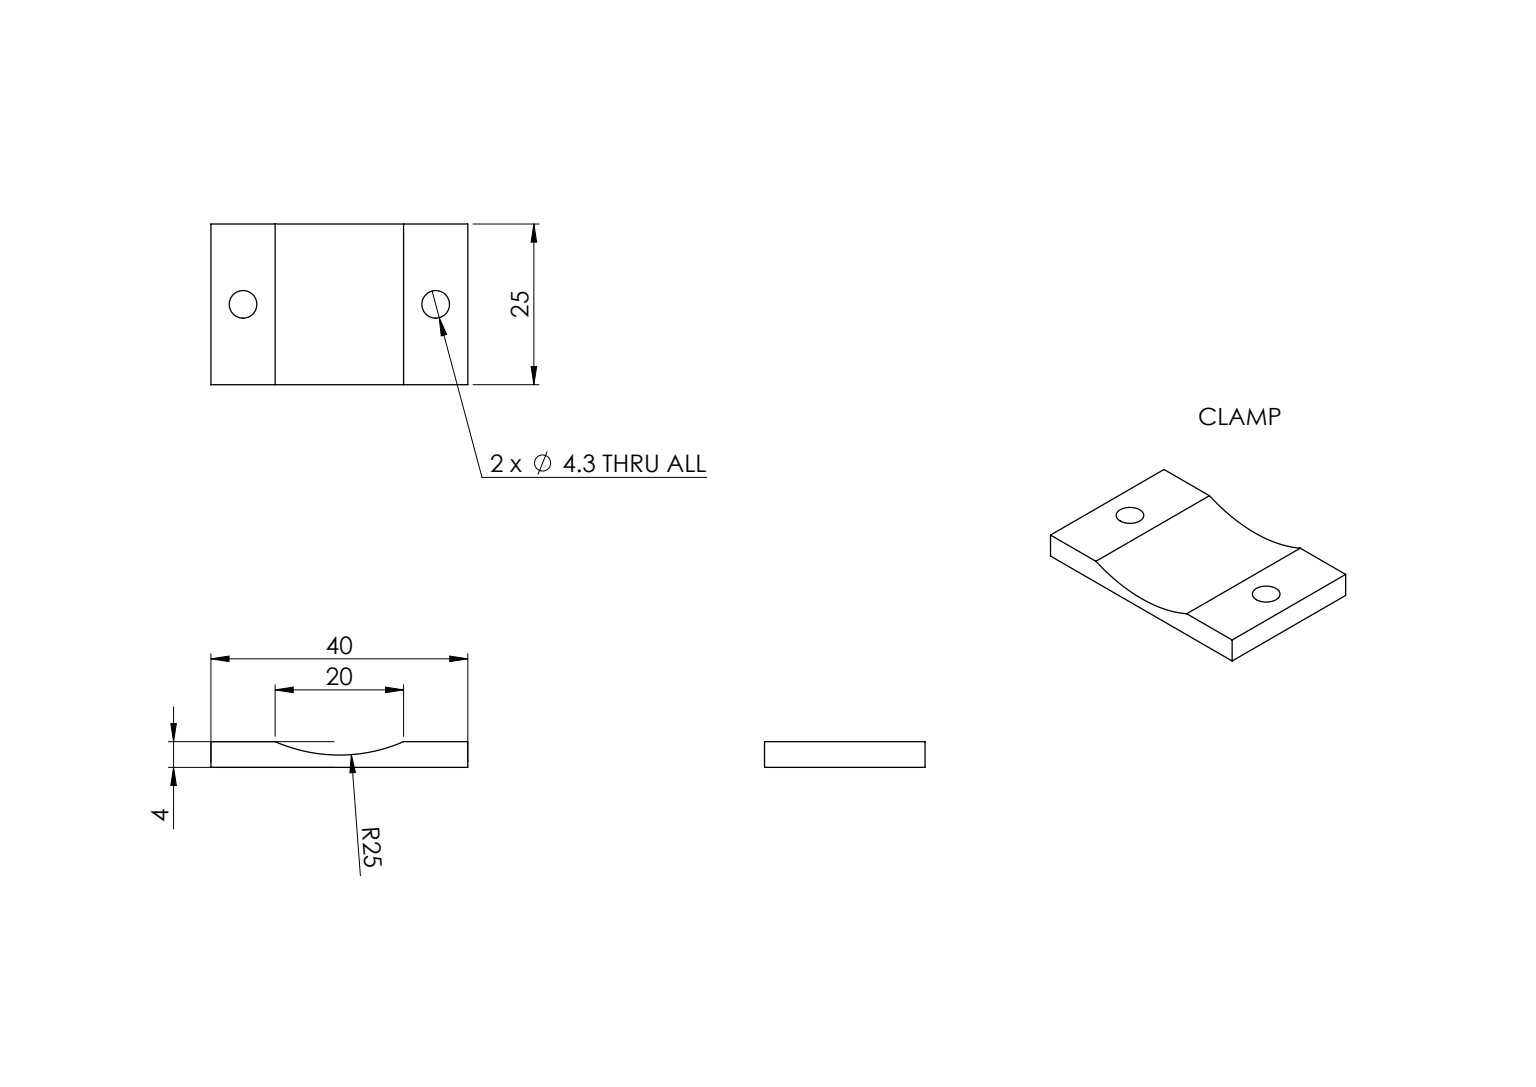
ISO-10303-21;
HEADER;
FILE_DESCRIPTION (('STEP AP214'),
    '1' );
FILE_NAME ('clamp.step',
    '2026-10-27T08:02:39',
    ( '' ),
    ( '' ),
    'SwSTEP 2.0',
    'SolidWorks 2026',
    '' );
FILE_SCHEMA (( 'AUTOMOTIVE_DESIGN' ));
ENDSEC;

DATA;
#6=PLANE ( 'NONE',  #3841 ) ;
#21=( GEOMETRIC_REPRESENTATION_CONTEXT ( 3 ) GLOBAL_UNCERTAINTY_ASSIGNED_CONTEXT ( ( #3529 ) ) GLOBAL_UNIT_ASSIGNED_CONTEXT ( ( #3001, #9758, #2180 ) ) REPRESENTATION_CONTEXT ( 'NONE', 'WORKASPACE' ) );
#33=SHAPE_DEFINITION_REPRESENTATION ( #1615, #7946 ) ;
#110=FACE_OUTER_BOUND ( 'NONE', #7615, .T. ) ;
#120=EDGE_LOOP ( 'NONE', ( #9318, #12086, #3898, #6255 ) ) ;
#123=ORIENTED_EDGE ( 'NONE', *, *, #7333, .T. ) ;
#156=ORIENTED_EDGE ( 'NONE', *, *, #8748, .T. ) ;
#164=CARTESIAN_POINT ( 'NONE',  ( 10.00000000000000000, 44.00000000000001421, -12.50000000000000000 ) ) ;
#182=SURFACE_STYLE_USAGE ( .BOTH. , #5944 ) ;
#191=EDGE_CURVE ( 'NONE', #922, #11041, #11147, .T. ) ;
#200=DIRECTION ( 'NONE',  ( 0.000000000000000000, 0.000000000000000000, 1.000000000000000000 ) ) ;
#212=CARTESIAN_POINT ( 'NONE',  ( 0.000000000000000000, 0.000000000000000000, 0.000000000000000000 ) ) ;
#250=FILL_AREA_STYLE ('',( #6001 ) ) ;
#268=LINE ( 'NONE', #2137, #3626 ) ;
#310=DIRECTION ( 'NONE',  ( 0.000000000000000000, 0.000000000000000000, 1.000000000000000000 ) ) ;
#380=AXIS2_PLACEMENT_3D ( 'NONE', #8436, #6808, #10487 ) ;
#381=ORIENTED_EDGE ( 'NONE', *, *, #191, .T. ) ;
#428=AXIS2_PLACEMENT_3D ( 'NONE', #10140, #7338, #1516 ) ;
#454=AXIS2_PLACEMENT_3D ( 'NONE', #10757, #4010, #11636 ) ;
#455=ORIENTED_EDGE ( 'NONE', *, *, #11034, .T. ) ;
#482=ORIENTED_EDGE ( 'NONE', *, *, #7502, .T. ) ;
#501=DIRECTION ( 'NONE',  ( -0.000000000000000000, 1.000000000000000000, -0.000000000000000000 ) ) ;
#540=ORIENTED_EDGE ( 'NONE', *, *, #2766, .F. ) ;
#557=CARTESIAN_POINT ( 'NONE',  ( -20.00000000000000000, 40.00000000000000711, 12.50000000000000000 ) ) ;
#575=LINE ( 'NONE', #164, #4417 ) ;
#622=LINE ( 'NONE', #3508, #9651 ) ;
#696=LINE ( 'NONE', #8326, #6294 ) ;
#751=DIRECTION ( 'NONE',  ( 0.000000000000000000, -1.000000000000000000, 0.000000000000000000 ) ) ;
#775=EDGE_CURVE ( 'NONE', #5859, #1347, #8071, .T. ) ;
#802=EDGE_LOOP ( 'NONE', ( #5664, #1167, #12118, #8865 ) ) ;
#827=CARTESIAN_POINT ( 'NONE',  ( -20.00000000000000000, 44.00000000000001421, -12.50000000000000000 ) ) ;
#833=EDGE_LOOP ( 'NONE', ( #9307, #5030, #4044, #11673 ) ) ;
#873=CARTESIAN_POINT ( 'NONE',  ( -20.00000000000000000, 44.00000000000001421, -12.50000000000000000 ) ) ;
#880=LINE ( 'NONE', #2008, #11470 ) ;
#922=VERTEX_POINT ( 'NONE', #4486 ) ;
#938=DIRECTION ( 'NONE',  ( 1.000000000000000000, 1.734723475976807094E-16, 0.000000000000000000 ) ) ;
#948=FACE_OUTER_BOUND ( 'NONE', #120, .T. ) ;
#958=LINE ( 'NONE', #4848, #8432 ) ;
#963=ORIENTED_EDGE ( 'NONE', *, *, #1656, .T. ) ;
#981=PLANE ( 'NONE',  #380 ) ;
#988=PLANE ( 'NONE',  #3703 ) ;
#1008=DIRECTION ( 'NONE',  ( 0.000000000000000000, 0.000000000000000000, -1.000000000000000000 ) ) ;
#1011=DIRECTION ( 'NONE',  ( -0.000000000000000000, 0.000000000000000000, -1.000000000000000000 ) ) ;
#1085=PLANE ( 'NONE',  #3231 ) ;
#1093=CARTESIAN_POINT ( 'NONE',  ( 15.00000000000000355, 44.00000000000001421, 2.149999999999999023 ) ) ;
#1104=EDGE_LOOP ( 'NONE', ( #1748, #5954 ) ) ;
#1106=LINE ( 'NONE', #4917, #10396 ) ;
#1119=EDGE_CURVE ( 'NONE', #1183, #3700, #1106, .T. ) ;
#1167=ORIENTED_EDGE ( 'NONE', *, *, #4711, .F. ) ;
#1183=VERTEX_POINT ( 'NONE', #2155 ) ;
#1197=CARTESIAN_POINT ( 'NONE',  ( -15.00000000000000000, 40.00000000000000711, -2.149999999999999023 ) ) ;
#1253=PRODUCT_DEFINITION_FORMATION_WITH_SPECIFIED_SOURCE ( 'ANY', '', #5415, .NOT_KNOWN. ) ;
#1276=DIRECTION ( 'NONE',  ( -0.000000000000000000, 1.000000000000000000, -0.000000000000000000 ) ) ;
#1281=CARTESIAN_POINT ( 'NONE',  ( -15.00000000000000000, 44.00000000000001421, 2.149999999999999023 ) ) ;
#1347=VERTEX_POINT ( 'NONE', #9237 ) ;
#1379=PRODUCT_DEFINITION_CONTEXT ( 'detailed design', #11353, 'design' ) ;
#1516=DIRECTION ( 'NONE',  ( 0.000000000000000000, 0.000000000000000000, 1.000000000000000000 ) ) ;
#1524=DIRECTION ( 'NONE',  ( 0.000000000000000000, 0.000000000000000000, 1.000000000000000000 ) ) ;
#1529=DIRECTION ( 'NONE',  ( -0.000000000000000000, -0.000000000000000000, -1.000000000000000000 ) ) ;
#1539=EDGE_LOOP ( 'NONE', ( #8919, #12318 ) ) ;
#1559=ORIENTED_EDGE ( 'NONE', *, *, #8748, .F. ) ;
#1615=PRODUCT_DEFINITION_SHAPE ( 'NONE', 'NONE',  #5170 ) ;
#1617=ORIENTED_EDGE ( 'NONE', *, *, #3552, .F. ) ;
#1626=CARTESIAN_POINT ( 'NONE',  ( -20.00000000000000000, 44.00000000000001421, 12.50000000000000000 ) ) ;
#1632=ORIENTED_EDGE ( 'NONE', *, *, #9751, .F. ) ;
#1656=EDGE_CURVE ( 'NONE', #5033, #7872, #6765, .T. ) ;
#1714=DIRECTION ( 'NONE',  ( -0.000000000000000000, 1.000000000000000000, -0.000000000000000000 ) ) ;
#1719=EDGE_CURVE ( 'NONE', #10717, #10090, #7363, .T. ) ;
#1739=DIRECTION ( 'NONE',  ( 0.000000000000000000, 0.000000000000000000, -1.000000000000000000 ) ) ;
#1748=ORIENTED_EDGE ( 'NONE', *, *, #4711, .T. ) ;
#1789=EDGE_CURVE ( 'NONE', #8068, #9485, #9216, .T. ) ;
#1851=CARTESIAN_POINT ( 'NONE',  ( 20.00000000000000000, 40.00000000000001421, 12.50000000000000000 ) ) ;
#1952=PLANE ( 'NONE',  #7605 ) ;
#1961=ADVANCED_FACE ( 'NONE', ( #10318 ), #1952, .F. ) ;
#1974=AXIS2_PLACEMENT_3D ( 'NONE', #6094, #1276, #5963 ) ;
#2008=CARTESIAN_POINT ( 'NONE',  ( -20.00000000000000000, 40.00000000000000711, 12.50000000000000000 ) ) ;
#2022=DIRECTION ( 'NONE',  ( 0.000000000000000000, 0.000000000000000000, 1.000000000000000000 ) ) ;
#2137=CARTESIAN_POINT ( 'NONE',  ( 20.00000000000000000, 44.00000000000002132, 12.50000000000000000 ) ) ;
#2155=CARTESIAN_POINT ( 'NONE',  ( -20.00000000000000000, 44.00000000000001421, 12.50000000000000000 ) ) ;
#2180=( NAMED_UNIT ( * ) SI_UNIT ( $, .STERADIAN. ) SOLID_ANGLE_UNIT ( ) );
#2209=DIRECTION ( 'NONE',  ( 0.000000000000000000, 0.000000000000000000, 1.000000000000000000 ) ) ;
#2227=FACE_OUTER_BOUND ( 'NONE', #833, .T. ) ;
#2254=AXIS2_PLACEMENT_3D ( 'NONE', #1626, #5448, #9269 ) ;
#2317=CARTESIAN_POINT ( 'NONE',  ( -3.469446951953614189E-15, 66.91287847477919115, 12.50000000000000000 ) ) ;
#2368=PLANE ( 'NONE',  #2254 ) ;
#2420=ORIENTED_EDGE ( 'NONE', *, *, #5139, .F. ) ;
#2445=DIRECTION ( 'NONE',  ( 0.000000000000000000, 0.000000000000000000, 1.000000000000000000 ) ) ;
#2483=VECTOR ( 'NONE', #4656, 1000.000000000000000 ) ;
#2494=ORIENTED_EDGE ( 'NONE', *, *, #11514, .F. ) ;
#2512=CARTESIAN_POINT ( 'NONE',  ( 20.00000000000000000, 44.00000000000002132, -12.50000000000000000 ) ) ;
#2546=ADVANCED_FACE ( 'NONE', ( #2227 ), #10729, .F. ) ;
#2558=ORIENTED_EDGE ( 'NONE', *, *, #191, .F. ) ;
#2577=CARTESIAN_POINT ( 'NONE',  ( 15.00000000000000355, 40.00000000000000711, 0.000000000000000000 ) ) ;
#2607=STYLED_ITEM('',(#12384),#8751);
#2633=VECTOR ( 'NONE', #4313, 1000.000000000000000 ) ;
#2695=AXIS2_PLACEMENT_3D ( 'NONE', #9940, #11549, #310 ) ;
#2736=ORIENTED_EDGE ( 'NONE', *, *, #3254, .T. ) ;
#2766=EDGE_CURVE ( 'NONE', #4747, #9384, #958, .T. ) ;
#2816=EDGE_CURVE ( 'NONE', #5214, #10090, #7674, .T. ) ;
#2820=APPLICATION_CONTEXT ( 'automotive_design' ) ;
#2833=MECHANICAL_DESIGN_GEOMETRIC_PRESENTATION_REPRESENTATION('',(#8831),#21);
#2860=CARTESIAN_POINT ( 'NONE',  ( -20.00000000000000000, 40.00000000000000711, -12.50000000000000000 ) ) ;
#2895=DIRECTION ( 'NONE',  ( -1.000000000000000000, 0.000000000000000000, -0.000000000000000000 ) ) ;
#2947=( NAMED_UNIT ( * ) SI_UNIT ( $, .STERADIAN. ) SOLID_ANGLE_UNIT ( ) );
#2973=VECTOR ( 'NONE', #6683, 1000.000000000000000 ) ;
#3001=( LENGTH_UNIT ( ) NAMED_UNIT ( * ) SI_UNIT ( .MILLI., .METRE. ) );
#3007=DIRECTION ( 'NONE',  ( -0.000000000000000000, 1.000000000000000000, -0.000000000000000000 ) ) ;
#3019=DIRECTION ( 'NONE',  ( -0.000000000000000000, 1.000000000000000000, -0.000000000000000000 ) ) ;
#3189=( NAMED_UNIT ( * ) SI_UNIT ( $, .STERADIAN. ) SOLID_ANGLE_UNIT ( ) );
#3231=AXIS2_PLACEMENT_3D ( 'NONE', #4896, #6847, #2022 ) ;
#3254=EDGE_CURVE ( 'NONE', #5033, #4657, #3760, .T. ) ;
#3285=AXIS2_PLACEMENT_3D ( 'NONE', #2577, #6288, #5402 ) ;
#3293=ORIENTED_EDGE ( 'NONE', *, *, #11266, .T. ) ;
#3310=CARTESIAN_POINT ( 'NONE',  ( -15.00000000000000000, 44.00000000000001421, 0.000000000000000000 ) ) ;
#3335=ADVANCED_FACE ( 'NONE', ( #11382 ), #6, .T. ) ;
#3396=DIRECTION ( 'NONE',  ( 1.000000000000000000, 0.000000000000000000, 0.000000000000000000 ) ) ;
#3434=VECTOR ( 'NONE', #6861, 1000.000000000000000 ) ;
#3508=CARTESIAN_POINT ( 'NONE',  ( 20.00000000000000000, 40.00000000000001421, 12.50000000000000000 ) ) ;
#3513=ORIENTED_EDGE ( 'NONE', *, *, #6548, .F. ) ;
#3514=DIRECTION ( 'NONE',  ( -1.000000000000000000, -1.734723475976807094E-16, 0.000000000000000000 ) ) ;
#3518=EDGE_CURVE ( 'NONE', #4612, #4657, #6859, .T. ) ;
#3528=CARTESIAN_POINT ( 'NONE',  ( 20.00000000000000000, 44.00000000000002132, 12.50000000000000000 ) ) ;
#3529=UNCERTAINTY_MEASURE_WITH_UNIT (LENGTH_MEASURE( 1.000000000000000082E-05 ), #3001, 'distance_accuracy_value', 'NONE');
#3552=EDGE_CURVE ( 'NONE', #9384, #9485, #622, .T. ) ;
#3571=FACE_BOUND ( 'NONE', #7648, .T. ) ;
#3580=ADVANCED_FACE ( 'NONE', ( #10183, #5378 ), #2368, .T. ) ;
#3585=FACE_OUTER_BOUND ( 'NONE', #802, .T. ) ;
#3626=VECTOR ( 'NONE', #5957, 1000.000000000000000 ) ;
#3643=EDGE_CURVE ( 'NONE', #7872, #5033, #11632, .T. ) ;
#3647=ORIENTED_EDGE ( 'NONE', *, *, #3552, .T. ) ;
#3700=VERTEX_POINT ( 'NONE', #873 ) ;
#3703=AXIS2_PLACEMENT_3D ( 'NONE', #10492, #1739, #9504 ) ;
#3714=LINE ( 'NONE', #8718, #2483 ) ;
#3760=LINE ( 'NONE', #9521, #6439 ) ;
#3773=AXIS2_PLACEMENT_3D ( 'NONE', #12073, #1524, #3396 ) ;
#3791=ORIENTED_EDGE ( 'NONE', *, *, #1789, .F. ) ;
#3841=AXIS2_PLACEMENT_3D ( 'NONE', #4704, #6657, #1011 ) ;
#3862=VERTEX_POINT ( 'NONE', #4933 ) ;
#3898=ORIENTED_EDGE ( 'NONE', *, *, #3518, .T. ) ;
#3997=FACE_OUTER_BOUND ( 'NONE', #10581, .T. ) ;
#4010=DIRECTION ( 'NONE',  ( -0.000000000000000000, 1.000000000000000000, -0.000000000000000000 ) ) ;
#4022=AXIS2_PLACEMENT_3D ( 'NONE', #5295, #8061, #7113 ) ;
#4035=DIRECTION ( 'NONE',  ( 0.000000000000000000, 0.000000000000000000, 1.000000000000000000 ) ) ;
#4044=ORIENTED_EDGE ( 'NONE', *, *, #775, .T. ) ;
#4089=DIRECTION ( 'NONE',  ( -0.000000000000000000, 1.000000000000000000, -0.000000000000000000 ) ) ;
#4313=DIRECTION ( 'NONE',  ( 0.000000000000000000, 1.000000000000000000, 0.000000000000000000 ) ) ;
#4417=VECTOR ( 'NONE', #8972, 1000.000000000000000 ) ;
#4451=CARTESIAN_POINT ( 'NONE',  ( -20.00000000000000000, 40.00000000000000711, 12.50000000000000000 ) ) ;
#4486=CARTESIAN_POINT ( 'NONE',  ( -20.00000000000000000, 40.00000000000000711, 12.50000000000000000 ) ) ;
#4524=ORIENTED_EDGE ( 'NONE', *, *, #1119, .F. ) ;
#4568=AXIS2_PLACEMENT_3D ( 'NONE', #8403, #6285, #7153 ) ;
#4579=CYLINDRICAL_SURFACE ( 'NONE', #4568, 2.149999999999999023 ) ;
#4612=VERTEX_POINT ( 'NONE', #6102 ) ;
#4654=DIRECTION ( 'NONE',  ( 1.000000000000000000, 1.734723475976807094E-16, 0.000000000000000000 ) ) ;
#4656=DIRECTION ( 'NONE',  ( 1.000000000000000000, 1.734723475976807094E-16, 0.000000000000000000 ) ) ;
#4657=VERTEX_POINT ( 'NONE', #1281 ) ;
#4704=CARTESIAN_POINT ( 'NONE',  ( 20.00000000000000000, 44.00000000000002132, 12.50000000000000000 ) ) ;
#4711=EDGE_CURVE ( 'NONE', #5214, #6431, #9677, .T. ) ;
#4747=VERTEX_POINT ( 'NONE', #3528 ) ;
#4776=DIRECTION ( 'NONE',  ( 0.000000000000000000, -1.000000000000000000, 0.000000000000000000 ) ) ;
#4791=EDGE_LOOP ( 'NONE', ( #3791, #6174, #10394, #3647 ) ) ;
#4848=CARTESIAN_POINT ( 'NONE',  ( 20.00000000000000000, 44.00000000000002132, 12.50000000000000000 ) ) ;
#4896=CARTESIAN_POINT ( 'NONE',  ( -20.00000000000000000, 40.00000000000000711, 12.50000000000000000 ) ) ;
#4917=CARTESIAN_POINT ( 'NONE',  ( -20.00000000000000000, 44.00000000000001421, 12.50000000000000000 ) ) ;
#4933=CARTESIAN_POINT ( 'NONE',  ( 10.00000000000000000, 44.00000000000001421, 12.50000000000000000 ) ) ;
#4936=EDGE_CURVE ( 'NONE', #11041, #9485, #3714, .T. ) ;
#5030=ORIENTED_EDGE ( 'NONE', *, *, #7502, .F. ) ;
#5033=VERTEX_POINT ( 'NONE', #5082 ) ;
#5082=CARTESIAN_POINT ( 'NONE',  ( -15.00000000000000000, 40.00000000000000711, 2.149999999999999023 ) ) ;
#5139=EDGE_CURVE ( 'NONE', #1183, #1347, #696, .T. ) ;
#5153=LINE ( 'NONE', #8982, #8591 ) ;
#5159=ADVANCED_FACE ( 'NONE', ( #8388, #3571, #9095 ), #7390, .F. ) ;
#5170=PRODUCT_DEFINITION ( 'UNKNOWN', '', #1253, #1379 ) ;
#5214=VERTEX_POINT ( 'NONE', #12180 ) ;
#5253=EDGE_CURVE ( 'NONE', #922, #9384, #880, .T. ) ;
#5295=CARTESIAN_POINT ( 'NONE',  ( -3.469446951953614189E-15, 66.91287847477919115, -12.50000000000000000 ) ) ;
#5321=DIRECTION ( 'NONE',  ( 0.000000000000000000, 0.000000000000000000, 1.000000000000000000 ) ) ;
#5330=CARTESIAN_POINT ( 'NONE',  ( 15.00000000000000355, 40.00000000000000711, -2.149999999999999023 ) ) ;
#5378=FACE_OUTER_BOUND ( 'NONE', #6865, .T. ) ;
#5384=DIRECTION ( 'NONE',  ( 1.000000000000000000, 1.734723475976807094E-16, 0.000000000000000000 ) ) ;
#5402=DIRECTION ( 'NONE',  ( 0.000000000000000000, 0.000000000000000000, 1.000000000000000000 ) ) ;
#5404=ORIENTED_EDGE ( 'NONE', *, *, #5253, .T. ) ;
#5415=PRODUCT ( 'clamp', 'clamp', '', ( #10409 ) ) ;
#5444=AXIS2_PLACEMENT_3D ( 'NONE', #5821, #10637, #6829 ) ;
#5448=DIRECTION ( 'NONE',  ( -1.734723475976807094E-16, 1.000000000000000000, 0.000000000000000000 ) ) ;
#5496=EDGE_CURVE ( 'NONE', #6431, #5214, #11481, .T. ) ;
#5551=FACE_OUTER_BOUND ( 'NONE', #5611, .T. ) ;
#5566=FACE_OUTER_BOUND ( 'NONE', #9905, .T. ) ;
#5579=LINE ( 'NONE', #827, #8418 ) ;
#5611=EDGE_LOOP ( 'NONE', ( #7612, #482, #3293, #7505, #6082, #9127 ) ) ;
#5623=CIRCLE ( 'NONE', #7430, 24.99999999999998579 ) ;
#5664=ORIENTED_EDGE ( 'NONE', *, *, #8242, .F. ) ;
#5683=LINE ( 'NONE', #8625, #6105 ) ;
#5726=ADVANCED_FACE ( 'NONE', ( #5551 ), #988, .T. ) ;
#5728=EDGE_CURVE ( 'NONE', #3700, #5859, #5683, .T. ) ;
#5796=DIRECTION ( 'NONE',  ( -0.000000000000000000, -0.000000000000000000, -1.000000000000000000 ) ) ;
#5821=CARTESIAN_POINT ( 'NONE',  ( 15.00000000000000355, 44.00000000000001421, 0.000000000000000000 ) ) ;
#5838=CYLINDRICAL_SURFACE ( 'NONE', #8037, 2.149999999999999023 ) ;
#5859=VERTEX_POINT ( 'NONE', #8744 ) ;
#5875=EDGE_LOOP ( 'NONE', ( #10517, #1617, #8585, #381 ) ) ;
#5944=SURFACE_SIDE_STYLE ('',( #9005 ) ) ;
#5954=ORIENTED_EDGE ( 'NONE', *, *, #5496, .T. ) ;
#5957=DIRECTION ( 'NONE',  ( -0.000000000000000000, -0.000000000000000000, -1.000000000000000000 ) ) ;
#5963=DIRECTION ( 'NONE',  ( 0.000000000000000000, 0.000000000000000000, 1.000000000000000000 ) ) ;
#6001=FILL_AREA_STYLE_COLOUR ( '', #11794 ) ;
#6056=AXIS2_PLACEMENT_3D ( 'NONE', #212, #4035, #8864 ) ;
#6082=ORIENTED_EDGE ( 'NONE', *, *, #4936, .F. ) ;
#6094=CARTESIAN_POINT ( 'NONE',  ( 15.00000000000000355, 44.00000000000001421, 0.000000000000000000 ) ) ;
#6102=CARTESIAN_POINT ( 'NONE',  ( -15.00000000000000000, 44.00000000000001421, -2.149999999999999023 ) ) ;
#6105=VECTOR ( 'NONE', #11236, 1000.000000000000000 ) ;
#6111=EDGE_LOOP ( 'NONE', ( #11130, #2420, #2494, #5404, #540, #1559 ) ) ;
#6173=DIRECTION ( 'NONE',  ( 0.000000000000000000, 0.000000000000000000, 1.000000000000000000 ) ) ;
#6174=ORIENTED_EDGE ( 'NONE', *, *, #11426, .F. ) ;
#6206=VECTOR ( 'NONE', #9576, 1000.000000000000000 ) ;
#6255=ORIENTED_EDGE ( 'NONE', *, *, #3254, .F. ) ;
#6265=DIRECTION ( 'NONE',  ( -0.000000000000000000, -0.000000000000000000, -1.000000000000000000 ) ) ;
#6271=DIRECTION ( 'NONE',  ( 1.000000000000000000, 0.000000000000000000, 0.000000000000000000 ) ) ;
#6285=DIRECTION ( 'NONE',  ( -0.000000000000000000, 1.000000000000000000, -0.000000000000000000 ) ) ;
#6288=DIRECTION ( 'NONE',  ( -0.000000000000000000, 1.000000000000000000, -0.000000000000000000 ) ) ;
#6294=VECTOR ( 'NONE', #5384, 1000.000000000000000 ) ;
#6392=ADVANCED_FACE ( 'NONE', ( #5566 ), #7461, .F. ) ;
#6431=VERTEX_POINT ( 'NONE', #5330 ) ;
#6439=VECTOR ( 'NONE', #9655, 1000.000000000000000 ) ;
#6478=CARTESIAN_POINT ( 'NONE',  ( -20.00000000000000000, 40.00000000000000711, 12.50000000000000000 ) ) ;
#6548=EDGE_CURVE ( 'NONE', #7872, #4612, #7761, .T. ) ;
#6573=AXIS2_PLACEMENT_3D ( 'NONE', #3310, #7121, #6173 ) ;
#6657=DIRECTION ( 'NONE',  ( 1.000000000000000000, 0.000000000000000000, -0.000000000000000000 ) ) ;
#6683=DIRECTION ( 'NONE',  ( 0.000000000000000000, 1.000000000000000000, 0.000000000000000000 ) ) ;
#6765=CIRCLE ( 'NONE', #8763, 2.149999999999999023 ) ;
#6766=( NAMED_UNIT ( * ) PLANE_ANGLE_UNIT ( ) SI_UNIT ( $, .RADIAN. ) );
#6808=DIRECTION ( 'NONE',  ( -1.734723475976807094E-16, 1.000000000000000000, 0.000000000000000000 ) ) ;
#6829=DIRECTION ( 'NONE',  ( 0.000000000000000000, 0.000000000000000000, 1.000000000000000000 ) ) ;
#6847=DIRECTION ( 'NONE',  ( -1.000000000000000000, 0.000000000000000000, 0.000000000000000000 ) ) ;
#6859=CIRCLE ( 'NONE', #454, 2.149999999999999023 ) ;
#6861=DIRECTION ( 'NONE',  ( -0.000000000000000000, 1.000000000000000000, -0.000000000000000000 ) ) ;
#6865=EDGE_LOOP ( 'NONE', ( #7868, #455, #156, #9120 ) ) ;
#7070=( NAMED_UNIT ( * ) PLANE_ANGLE_UNIT ( ) SI_UNIT ( $, .RADIAN. ) );
#7113=DIRECTION ( 'NONE',  ( 1.000000000000000000, 0.000000000000000000, 0.000000000000000000 ) ) ;
#7121=DIRECTION ( 'NONE',  ( -0.000000000000000000, 1.000000000000000000, -0.000000000000000000 ) ) ;
#7153=DIRECTION ( 'NONE',  ( 0.000000000000000000, 0.000000000000000000, 1.000000000000000000 ) ) ;
#7176=CIRCLE ( 'NONE', #6573, 2.149999999999999023 ) ;
#7184=VERTEX_POINT ( 'NONE', #8995 ) ;
#7218=CARTESIAN_POINT ( 'NONE',  ( 15.00000000000000355, 44.00000000000001421, 0.000000000000000000 ) ) ;
#7280=EDGE_LOOP ( 'NONE', ( #9283, #2558, #7683, #8728 ) ) ;
#7333=EDGE_CURVE ( 'NONE', #4657, #4612, #7176, .T. ) ;
#7338=DIRECTION ( 'NONE',  ( -0.000000000000000000, 1.000000000000000000, -0.000000000000000000 ) ) ;
#7363=CIRCLE ( 'NONE', #1974, 2.149999999999999023 ) ;
#7368=ORIENTED_EDGE ( 'NONE', *, *, #2816, .F. ) ;
#7390=PLANE ( 'NONE',  #10479 ) ;
#7430=AXIS2_PLACEMENT_3D ( 'NONE', #2317, #2445, #6271 ) ;
#7458=EDGE_CURVE ( 'NONE', #11041, #3700, #10291, .T. ) ;
#7461=CYLINDRICAL_SURFACE ( 'NONE', #428, 2.149999999999999023 ) ;
#7502=EDGE_CURVE ( 'NONE', #5859, #7184, #10763, .T. ) ;
#7505=ORIENTED_EDGE ( 'NONE', *, *, #1789, .T. ) ;
#7515=ORIENTED_EDGE ( 'NONE', *, *, #1656, .F. ) ;
#7539=ADVANCED_FACE ( 'NONE', ( #3585 ), #4579, .F. ) ;
#7605=AXIS2_PLACEMENT_3D ( 'NONE', #8650, #1008, #2895 ) ;
#7612=ORIENTED_EDGE ( 'NONE', *, *, #5728, .T. ) ;
#7615=EDGE_LOOP ( 'NONE', ( #7956, #7678, #4524, #8199 ) ) ;
#7648=EDGE_LOOP ( 'NONE', ( #963, #9503 ) ) ;
#7652=CIRCLE ( 'NONE', #9846, 2.149999999999999023 ) ;
#7674=LINE ( 'NONE', #1093, #3434 ) ;
#7678=ORIENTED_EDGE ( 'NONE', *, *, #5728, .F. ) ;
#7683=ORIENTED_EDGE ( 'NONE', *, *, #11514, .T. ) ;
#7761=LINE ( 'NONE', #10378, #11166 ) ;
#7823=SHAPE_REPRESENTATION_RELATIONSHIP ( 'NONE' , 'NONE' ,  #7946, #11675 ) ;
#7858=AXIS2_PLACEMENT_3D ( 'NONE', #9089, #501, #5321 ) ;
#7868=ORIENTED_EDGE ( 'NONE', *, *, #11266, .F. ) ;
#7872=VERTEX_POINT ( 'NONE', #1197 ) ;
#7946=SHAPE_REPRESENTATION ( 'clamp', ( #6056 ), #12194 ) ;
#7956=ORIENTED_EDGE ( 'NONE', *, *, #775, .F. ) ;
#7997=VECTOR ( 'NONE', #8181, 1000.000000000000000 ) ;
#8003=( LENGTH_UNIT ( ) NAMED_UNIT ( * ) SI_UNIT ( .MILLI., .METRE. ) );
#8037=AXIS2_PLACEMENT_3D ( 'NONE', #11564, #3019, #200 ) ;
#8047=EDGE_LOOP ( 'NONE', ( #1632, #9661 ) ) ;
#8049=CARTESIAN_POINT ( 'NONE',  ( -20.00000000000000000, 40.00000000000000711, -12.50000000000000000 ) ) ;
#8061=DIRECTION ( 'NONE',  ( -0.000000000000000000, -0.000000000000000000, 1.000000000000000000 ) ) ;
#8068=VERTEX_POINT ( 'NONE', #9738 ) ;
#8071=LINE ( 'NONE', #11791, #7997 ) ;
#8181=DIRECTION ( 'NONE',  ( -0.000000000000000000, -0.000000000000000000, 1.000000000000000000 ) ) ;
#8199=ORIENTED_EDGE ( 'NONE', *, *, #5139, .T. ) ;
#8242=EDGE_CURVE ( 'NONE', #6431, #10717, #5153, .T. ) ;
#8326=CARTESIAN_POINT ( 'NONE',  ( -20.00000000000000000, 44.00000000000001421, 12.50000000000000000 ) ) ;
#8376=VECTOR ( 'NONE', #1529, 1000.000000000000000 ) ;
#8388=FACE_BOUND ( 'NONE', #1104, .T. ) ;
#8403=CARTESIAN_POINT ( 'NONE',  ( 15.00000000000000355, 44.00000000000001421, 0.000000000000000000 ) ) ;
#8418=VECTOR ( 'NONE', #4654, 1000.000000000000000 ) ;
#8432=VECTOR ( 'NONE', #4776, 1000.000000000000000 ) ;
#8436=CARTESIAN_POINT ( 'NONE',  ( -20.00000000000000000, 44.00000000000001421, 12.50000000000000000 ) ) ;
#8481=CARTESIAN_POINT ( 'NONE',  ( 20.00000000000000000, 40.00000000000001421, -12.50000000000000000 ) ) ;
#8585=ORIENTED_EDGE ( 'NONE', *, *, #5253, .F. ) ;
#8591=VECTOR ( 'NONE', #1714, 1000.000000000000000 ) ;
#8625=CARTESIAN_POINT ( 'NONE',  ( -20.00000000000000000, 44.00000000000001421, -12.50000000000000000 ) ) ;
#8649=LINE ( 'NONE', #10453, #6206 ) ;
#8650=CARTESIAN_POINT ( 'NONE',  ( 0.000000000000000000, 0.000000000000000000, 12.50000000000000000 ) ) ;
#8660=UNCERTAINTY_MEASURE_WITH_UNIT (LENGTH_MEASURE( 1.000000000000000082E-05 ), #8708, 'distance_accuracy_value', 'NONE');
#8686=FACE_BOUND ( 'NONE', #1539, .T. ) ;
#8708=( LENGTH_UNIT ( ) NAMED_UNIT ( * ) SI_UNIT ( .MILLI., .METRE. ) );
#8718=CARTESIAN_POINT ( 'NONE',  ( -20.00000000000000000, 40.00000000000000711, -12.50000000000000000 ) ) ;
#8728=ORIENTED_EDGE ( 'NONE', *, *, #1119, .T. ) ;
#8744=CARTESIAN_POINT ( 'NONE',  ( -10.00000000000000000, 44.00000000000001421, -12.50000000000000000 ) ) ;
#8748=EDGE_CURVE ( 'NONE', #3862, #4747, #8649, .T. ) ;
#8751=MANIFOLD_SOLID_BREP ( 'M4 Clearance Hole1', #8781 ) ;
#8763=AXIS2_PLACEMENT_3D ( 'NONE', #8966, #11701, #10771 ) ;
#8781=CLOSED_SHELL ( 'NONE', ( #11754, #11345, #3580, #1961, #5726, #5159, #3335, #10839, #11328, #2546, #6392, #7539 ) ) ;
#8811=( GEOMETRIC_REPRESENTATION_CONTEXT ( 3 ) GLOBAL_UNCERTAINTY_ASSIGNED_CONTEXT ( ( #8660 ) ) GLOBAL_UNIT_ASSIGNED_CONTEXT ( ( #8708, #6766, #2947 ) ) REPRESENTATION_CONTEXT ( 'NONE', 'WORKASPACE' ) );
#8831=STYLED_ITEM ( 'NONE', ( #8945 ), #11675 ) ;
#8864=DIRECTION ( 'NONE',  ( 1.000000000000000000, 0.000000000000000000, 0.000000000000000000 ) ) ;
#8865=ORIENTED_EDGE ( 'NONE', *, *, #9751, .T. ) ;
#8883=ORIENTED_EDGE ( 'NONE', *, *, #5496, .F. ) ;
#8919=ORIENTED_EDGE ( 'NONE', *, *, #7333, .F. ) ;
#8945=PRESENTATION_STYLE_ASSIGNMENT (( #182 ) ) ;
#8966=CARTESIAN_POINT ( 'NONE',  ( -15.00000000000000000, 40.00000000000000711, 0.000000000000000000 ) ) ;
#8972=DIRECTION ( 'NONE',  ( -0.000000000000000000, -0.000000000000000000, 1.000000000000000000 ) ) ;
#8982=CARTESIAN_POINT ( 'NONE',  ( 15.00000000000000355, 44.00000000000001421, -2.149999999999999023 ) ) ;
#8995=CARTESIAN_POINT ( 'NONE',  ( 10.00000000000000711, 44.00000000000001421, -12.50000000000000000 ) ) ;
#9005=SURFACE_STYLE_FILL_AREA ( #250 ) ;
#9014=MECHANICAL_DESIGN_GEOMETRIC_PRESENTATION_REPRESENTATION('',(#2607),#8811);
#9089=CARTESIAN_POINT ( 'NONE',  ( -15.00000000000000000, 40.00000000000000711, 0.000000000000000000 ) ) ;
#9095=FACE_OUTER_BOUND ( 'NONE', #5875, .T. ) ;
#9120=ORIENTED_EDGE ( 'NONE', *, *, #11426, .T. ) ;
#9127=ORIENTED_EDGE ( 'NONE', *, *, #7458, .T. ) ;
#9216=LINE ( 'NONE', #2512, #12133 ) ;
#9237=CARTESIAN_POINT ( 'NONE',  ( -10.00000000000000000, 44.00000000000001421, 12.50000000000000000 ) ) ;
#9269=DIRECTION ( 'NONE',  ( -1.000000000000000000, -1.734723475976807094E-16, 0.000000000000000000 ) ) ;
#9283=ORIENTED_EDGE ( 'NONE', *, *, #7458, .F. ) ;
#9307=ORIENTED_EDGE ( 'NONE', *, *, #11034, .F. ) ;
#9318=ORIENTED_EDGE ( 'NONE', *, *, #3643, .F. ) ;
#9384=VERTEX_POINT ( 'NONE', #1851 ) ;
#9485=VERTEX_POINT ( 'NONE', #8481 ) ;
#9494=ORIENTED_EDGE ( 'NONE', *, *, #1719, .T. ) ;
#9503=ORIENTED_EDGE ( 'NONE', *, *, #3643, .T. ) ;
#9504=DIRECTION ( 'NONE',  ( -1.000000000000000000, 0.000000000000000000, -0.000000000000000000 ) ) ;
#9521=CARTESIAN_POINT ( 'NONE',  ( -15.00000000000000000, 44.00000000000001421, 2.149999999999999023 ) ) ;
#9524=FACE_OUTER_BOUND ( 'NONE', #7280, .T. ) ;
#9576=DIRECTION ( 'NONE',  ( 1.000000000000000000, 1.734723475976807094E-16, 0.000000000000000000 ) ) ;
#9651=VECTOR ( 'NONE', #6265, 1000.000000000000000 ) ;
#9655=DIRECTION ( 'NONE',  ( -0.000000000000000000, 1.000000000000000000, -0.000000000000000000 ) ) ;
#9661=ORIENTED_EDGE ( 'NONE', *, *, #1719, .F. ) ;
#9677=CIRCLE ( 'NONE', #3285, 2.149999999999999023 ) ;
#9738=CARTESIAN_POINT ( 'NONE',  ( 20.00000000000000000, 44.00000000000002132, -12.50000000000000000 ) ) ;
#9751=EDGE_CURVE ( 'NONE', #10090, #10717, #7652, .T. ) ;
#9758=( NAMED_UNIT ( * ) PLANE_ANGLE_UNIT ( ) SI_UNIT ( $, .RADIAN. ) );
#9846=AXIS2_PLACEMENT_3D ( 'NONE', #7218, #4089, #2209 ) ;
#9905=EDGE_LOOP ( 'NONE', ( #3513, #7515, #2736, #123 ) ) ;
#9940=CARTESIAN_POINT ( 'NONE',  ( 15.00000000000000355, 40.00000000000000711, 0.000000000000000000 ) ) ;
#9951=LINE ( 'NONE', #557, #2633 ) ;
#10090=VERTEX_POINT ( 'NONE', #11813 ) ;
#10140=CARTESIAN_POINT ( 'NONE',  ( -15.00000000000000000, 44.00000000000001421, 0.000000000000000000 ) ) ;
#10183=FACE_BOUND ( 'NONE', #8047, .T. ) ;
#10291=LINE ( 'NONE', #2860, #2973 ) ;
#10318=FACE_OUTER_BOUND ( 'NONE', #6111, .T. ) ;
#10378=CARTESIAN_POINT ( 'NONE',  ( -15.00000000000000000, 44.00000000000001421, -2.149999999999999023 ) ) ;
#10393=UNCERTAINTY_MEASURE_WITH_UNIT (LENGTH_MEASURE( 1.000000000000000082E-05 ), #8003, 'distance_accuracy_value', 'NONE');
#10394=ORIENTED_EDGE ( 'NONE', *, *, #2766, .T. ) ;
#10396=VECTOR ( 'NONE', #5796, 1000.000000000000000 ) ;
#10409=PRODUCT_CONTEXT ( 'NONE', #2820, 'mechanical' ) ;
#10453=CARTESIAN_POINT ( 'NONE',  ( -20.00000000000000000, 44.00000000000001421, 12.50000000000000000 ) ) ;
#10479=AXIS2_PLACEMENT_3D ( 'NONE', #4451, #11186, #3514 ) ;
#10487=DIRECTION ( 'NONE',  ( -1.000000000000000000, -1.734723475976807094E-16, 0.000000000000000000 ) ) ;
#10492=CARTESIAN_POINT ( 'NONE',  ( 0.000000000000000000, 0.000000000000000000, -12.50000000000000000 ) ) ;
#10517=ORIENTED_EDGE ( 'NONE', *, *, #4936, .T. ) ;
#10581=EDGE_LOOP ( 'NONE', ( #8883, #11404, #9494, #7368 ) ) ;
#10637=DIRECTION ( 'NONE',  ( -0.000000000000000000, 1.000000000000000000, -0.000000000000000000 ) ) ;
#10696=CYLINDRICAL_SURFACE ( 'NONE', #5444, 2.149999999999999023 ) ;
#10717=VERTEX_POINT ( 'NONE', #11239 ) ;
#10729=CYLINDRICAL_SURFACE ( 'NONE', #4022, 24.99999999999998579 ) ;
#10757=CARTESIAN_POINT ( 'NONE',  ( -15.00000000000000000, 44.00000000000001421, 0.000000000000000000 ) ) ;
#10763=CIRCLE ( 'NONE', #3773, 24.99999999999998579 ) ;
#10771=DIRECTION ( 'NONE',  ( 0.000000000000000000, 0.000000000000000000, 1.000000000000000000 ) ) ;
#10839=ADVANCED_FACE ( 'NONE', ( #8686, #110 ), #981, .T. ) ;
#11034=EDGE_CURVE ( 'NONE', #7184, #3862, #575, .T. ) ;
#11041=VERTEX_POINT ( 'NONE', #8049 ) ;
#11130=ORIENTED_EDGE ( 'NONE', *, *, #11555, .F. ) ;
#11147=LINE ( 'NONE', #6478, #8376 ) ;
#11166=VECTOR ( 'NONE', #3007, 1000.000000000000000 ) ;
#11186=DIRECTION ( 'NONE',  ( -1.734723475976807094E-16, 1.000000000000000000, 0.000000000000000000 ) ) ;
#11236=DIRECTION ( 'NONE',  ( 1.000000000000000000, 1.734723475976807094E-16, 0.000000000000000000 ) ) ;
#11239=CARTESIAN_POINT ( 'NONE',  ( 15.00000000000000355, 44.00000000000001421, -2.149999999999999023 ) ) ;
#11266=EDGE_CURVE ( 'NONE', #7184, #8068, #5579, .T. ) ;
#11328=ADVANCED_FACE ( 'NONE', ( #9524 ), #1085, .T. ) ;
#11345=ADVANCED_FACE ( 'NONE', ( #948 ), #5838, .F. ) ;
#11353=APPLICATION_CONTEXT ( 'automotive_design' ) ;
#11382=FACE_OUTER_BOUND ( 'NONE', #4791, .T. ) ;
#11404=ORIENTED_EDGE ( 'NONE', *, *, #8242, .T. ) ;
#11426=EDGE_CURVE ( 'NONE', #4747, #8068, #268, .T. ) ;
#11470=VECTOR ( 'NONE', #938, 1000.000000000000000 ) ;
#11481=CIRCLE ( 'NONE', #2695, 2.149999999999999023 ) ;
#11514=EDGE_CURVE ( 'NONE', #922, #1183, #9951, .T. ) ;
#11549=DIRECTION ( 'NONE',  ( -0.000000000000000000, 1.000000000000000000, -0.000000000000000000 ) ) ;
#11555=EDGE_CURVE ( 'NONE', #1347, #3862, #5623, .T. ) ;
#11564=CARTESIAN_POINT ( 'NONE',  ( -15.00000000000000000, 44.00000000000001421, 0.000000000000000000 ) ) ;
#11632=CIRCLE ( 'NONE', #7858, 2.149999999999999023 ) ;
#11636=DIRECTION ( 'NONE',  ( 0.000000000000000000, 0.000000000000000000, 1.000000000000000000 ) ) ;
#11673=ORIENTED_EDGE ( 'NONE', *, *, #11555, .T. ) ;
#11675=ADVANCED_BREP_SHAPE_REPRESENTATION ( '', ( #8751, #6056 ), #12194 ) ;
#11701=DIRECTION ( 'NONE',  ( -0.000000000000000000, 1.000000000000000000, -0.000000000000000000 ) ) ;
#11754=ADVANCED_FACE ( 'NONE', ( #3997 ), #10696, .F. ) ;
#11791=CARTESIAN_POINT ( 'NONE',  ( -10.00000000000000000, 44.00000000000001421, -12.50000000000000000 ) ) ;
#11794=COLOUR_RGB ( '',0.8941176470588234615, 0.8941176470588234615, 0.8941176470588234615 ) ;
#11813=CARTESIAN_POINT ( 'NONE',  ( 15.00000000000000355, 44.00000000000001421, 2.149999999999999023 ) ) ;
#12073=CARTESIAN_POINT ( 'NONE',  ( -3.469446951953614189E-15, 66.91287847477919115, -12.50000000000000000 ) ) ;
#12086=ORIENTED_EDGE ( 'NONE', *, *, #6548, .T. ) ;
#12118=ORIENTED_EDGE ( 'NONE', *, *, #2816, .T. ) ;
#12133=VECTOR ( 'NONE', #751, 1000.000000000000000 ) ;
#12180=CARTESIAN_POINT ( 'NONE',  ( 15.00000000000000355, 40.00000000000000711, 2.149999999999999023 ) ) ;
#12194=( GEOMETRIC_REPRESENTATION_CONTEXT ( 3 ) GLOBAL_UNCERTAINTY_ASSIGNED_CONTEXT ( ( #10393 ) ) GLOBAL_UNIT_ASSIGNED_CONTEXT ( ( #8003, #7070, #3189 ) ) REPRESENTATION_CONTEXT ( 'NONE', 'WORKASPACE' ) );
#12318=ORIENTED_EDGE ( 'NONE', *, *, #3518, .F. ) ;
#12378=COLOUR_RGB('Light Blue',0.38,0.62,0.78);
#12379=FILL_AREA_STYLE_COLOUR('',#12378);
#12380=FILL_AREA_STYLE('',(#12379));
#12381=SURFACE_STYLE_FILL_AREA(#12380);
#12382=SURFACE_SIDE_STYLE('',(#12381));
#12383=SURFACE_STYLE_USAGE(.BOTH.,#12382);
#12384=PRESENTATION_STYLE_ASSIGNMENT((#12383));
ENDSEC;
END-ISO-10303-21;
